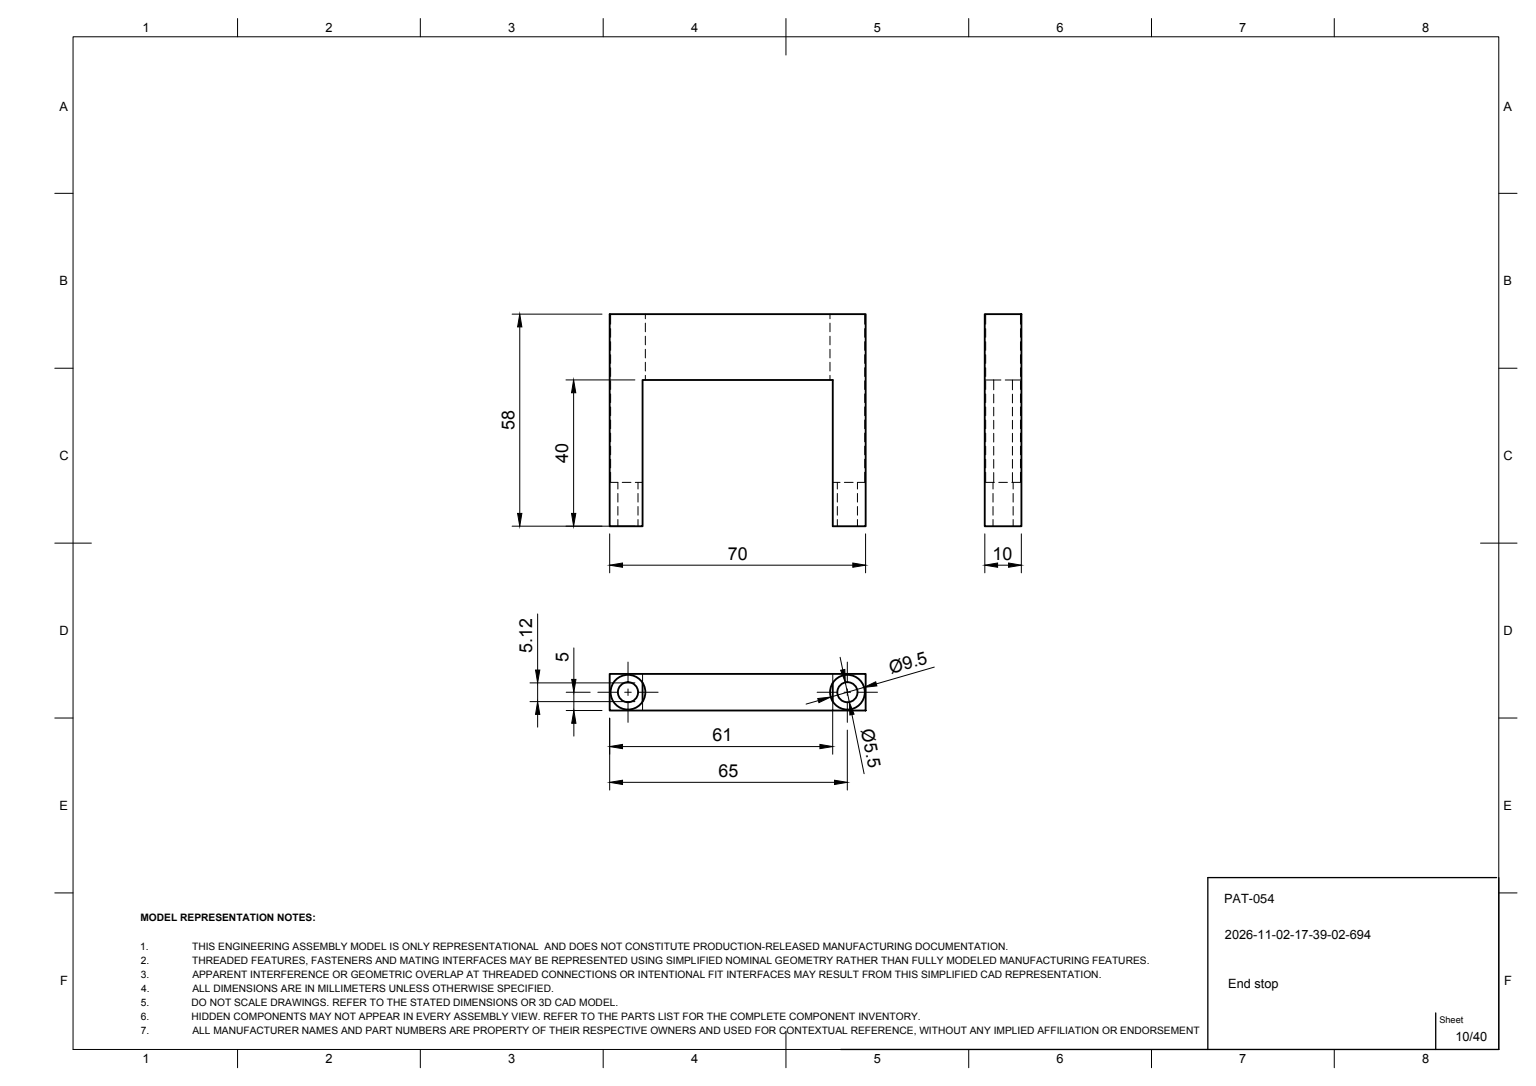
ISO-10303-21;
HEADER;
/* Generated by software containing ST-Developer
 * from STEP Tools, Inc. (www.steptools.com) 
 */

FILE_DESCRIPTION(
/* description */ ('PAT-054'),
/* implementation_level */ '2;1');

FILE_NAME(
/* name */ 'End stop.step',
/* time_stamp */ '2026-10-29T16:38:13-07:00',
/* author */ (''),
/* organization */ (''),
/* preprocessor_version */ 'ST-DEVELOPER v20.2',
/* originating_system */ 'Autodesk Translation Framework v15.17.0.0',
/* authorisation */ '');

FILE_SCHEMA (('AUTOMOTIVE_DESIGN { 1 0 10303 214 3 1 1 }'));
ENDSEC;

DATA;
#10=MECHANICAL_DESIGN_GEOMETRIC_PRESENTATION_REPRESENTATION('',(#905),#33981);
#817=SHAPE_REPRESENTATION_RELATIONSHIP('SRR','None',#34190,#861);
#861=ADVANCED_BREP_SHAPE_REPRESENTATION('',(#964),#33938);
#905=STYLED_ITEM('',(#34510),#964);
#964=MANIFOLD_SOLID_BREP('Body1',#13016);
#1104=FACE_BOUND('',#2486,.T.);
#1105=FACE_BOUND('',#2489,.T.);
#1106=FACE_BOUND('',#2498,.T.);
#1107=FACE_BOUND('',#2503,.T.);
#1108=FACE_BOUND('',#2504,.T.);
#1109=FACE_BOUND('',#2506,.T.);
#1269=PLANE('',#13771);
#1270=PLANE('',#13778);
#1271=PLANE('',#13785);
#1272=PLANE('',#13786);
#1273=PLANE('',#13791);
#1274=PLANE('',#13792);
#1275=PLANE('',#13793);
#1276=PLANE('',#13794);
#1277=PLANE('',#13795);
#1278=PLANE('',#13796);
#1279=PLANE('',#13797);
#1280=PLANE('',#13798);
#1670=FACE_OUTER_BOUND('',#2485,.T.);
#1671=FACE_OUTER_BOUND('',#2487,.T.);
#1672=FACE_OUTER_BOUND('',#2488,.T.);
#1673=FACE_OUTER_BOUND('',#2490,.T.);
#1674=FACE_OUTER_BOUND('',#2491,.T.);
#1675=FACE_OUTER_BOUND('',#2492,.T.);
#1676=FACE_OUTER_BOUND('',#2493,.T.);
#1677=FACE_OUTER_BOUND('',#2494,.T.);
#1678=FACE_OUTER_BOUND('',#2495,.T.);
#1679=FACE_OUTER_BOUND('',#2496,.T.);
#1680=FACE_OUTER_BOUND('',#2497,.T.);
#1681=FACE_OUTER_BOUND('',#2499,.T.);
#1682=FACE_OUTER_BOUND('',#2500,.T.);
#1683=FACE_OUTER_BOUND('',#2501,.T.);
#1684=FACE_OUTER_BOUND('',#2502,.T.);
#1685=FACE_OUTER_BOUND('',#2505,.T.);
#2485=EDGE_LOOP('',(#8915,#8916,#8917));
#2486=EDGE_LOOP('',(#8918));
#2487=EDGE_LOOP('',(#8919,#8920,#8921,#8922,#8923,#8924,#8925,#8926));
#2488=EDGE_LOOP('',(#8927,#8928,#8929));
#2489=EDGE_LOOP('',(#8930));
#2490=EDGE_LOOP('',(#8931,#8932,#8933,#8934,#8935,#8936,#8937,#8938));
#2491=EDGE_LOOP('',(#8939,#8940,#8941,#8942,#8943,#8944,#8945,#8946));
#2492=EDGE_LOOP('',(#8947,#8948,#8949,#8950,#8951,#8952,#8953,#8954));
#2493=EDGE_LOOP('',(#8955,#8956,#8957,#8958));
#2494=EDGE_LOOP('',(#8959,#8960,#8961,#8962));
#2495=EDGE_LOOP('',(#8963,#8964,#8965,#8966,#8967,#8968,#8969,#8970));
#2496=EDGE_LOOP('',(#8971,#8972,#8973,#8974,#8975,#8976,#8977,#8978));
#2497=EDGE_LOOP('',(#8979,#8980,#8981,#8982));
#2498=EDGE_LOOP('',(#8983));
#2499=EDGE_LOOP('',(#8984,#8985,#8986,#8987));
#2500=EDGE_LOOP('',(#8988,#8989,#8990,#8991));
#2501=EDGE_LOOP('',(#8992,#8993,#8994,#8995,#8996,#8997,#8998,#8999));
#2502=EDGE_LOOP('',(#9000,#9001,#9002,#9003));
#2503=EDGE_LOOP('',(#9004));
#2504=EDGE_LOOP('',(#9005));
#2505=EDGE_LOOP('',(#9006,#9007,#9008,#9009));
#2506=EDGE_LOOP('',(#9010));
#3342=LINE('',#18948,#4276);
#3343=LINE('',#18956,#4277);
#3344=LINE('',#18959,#4278);
#3345=LINE('',#18961,#4279);
#3346=LINE('',#18966,#4280);
#3347=LINE('',#18974,#4281);
#3348=LINE('',#18977,#4282);
#3349=LINE('',#18979,#4283);
#3350=LINE('',#18983,#4284);
#3351=LINE('',#18985,#4285);
#3352=LINE('',#18987,#4286);
#3353=LINE('',#18989,#4287);
#3354=LINE('',#18990,#4288);
#3355=LINE('',#18993,#4289);
#3356=LINE('',#18995,#4290);
#3357=LINE('',#18997,#4291);
#3358=LINE('',#18999,#4292);
#3359=LINE('',#19000,#4293);
#3360=LINE('',#19004,#4294);
#3361=LINE('',#19008,#4295);
#3362=LINE('',#19010,#4296);
#3363=LINE('',#19011,#4297);
#3364=LINE('',#19014,#4298);
#3365=LINE('',#19016,#4299);
#3366=LINE('',#19018,#4300);
#3367=LINE('',#19020,#4301);
#3368=LINE('',#19021,#4302);
#3369=LINE('',#19024,#4303);
#3370=LINE('',#19025,#4304);
#3371=LINE('',#19028,#4305);
#3372=LINE('',#19029,#4306);
#3373=LINE('',#19032,#4307);
#3374=LINE('',#19034,#4308);
#3375=LINE('',#19035,#4309);
#3376=LINE('',#19037,#4310);
#3377=LINE('',#19038,#4311);
#4276=VECTOR('',#15421,1.);
#4277=VECTOR('',#15430,1.);
#4278=VECTOR('',#15433,1.);
#4279=VECTOR('',#15434,0.475);
#4280=VECTOR('',#15439,1.);
#4281=VECTOR('',#15448,1.);
#4282=VECTOR('',#15451,1.);
#4283=VECTOR('',#15452,0.475);
#4284=VECTOR('',#15457,1.);
#4285=VECTOR('',#15458,1.);
#4286=VECTOR('',#15459,1.);
#4287=VECTOR('',#15460,1.);
#4288=VECTOR('',#15461,1.);
#4289=VECTOR('',#15464,1.);
#4290=VECTOR('',#15465,1.);
#4291=VECTOR('',#15466,1.);
#4292=VECTOR('',#15467,1.);
#4293=VECTOR('',#15468,1.);
#4294=VECTOR('',#15473,0.275);
#4295=VECTOR('',#15478,0.275);
#4296=VECTOR('',#15481,1.);
#4297=VECTOR('',#15482,1.);
#4298=VECTOR('',#15485,1.);
#4299=VECTOR('',#15486,1.);
#4300=VECTOR('',#15487,1.);
#4301=VECTOR('',#15488,1.);
#4302=VECTOR('',#15489,1.);
#4303=VECTOR('',#15492,1.);
#4304=VECTOR('',#15493,1.);
#4305=VECTOR('',#15496,1.);
#4306=VECTOR('',#15497,1.);
#4307=VECTOR('',#15500,1.);
#4308=VECTOR('',#15501,1.);
#4309=VECTOR('',#15502,1.);
#4310=VECTOR('',#15505,1.);
#4311=VECTOR('',#15506,1.);
#5213=CIRCLE('',#13772,0.475);
#5214=CIRCLE('',#13773,0.475);
#5215=CIRCLE('',#13774,0.275);
#5216=CIRCLE('',#13776,0.475);
#5217=CIRCLE('',#13777,0.475);
#5218=CIRCLE('',#13779,0.475);
#5219=CIRCLE('',#13780,0.475);
#5220=CIRCLE('',#13781,0.275);
#5221=CIRCLE('',#13783,0.475);
#5222=CIRCLE('',#13784,0.475);
#5223=CIRCLE('',#13788,0.275);
#5224=CIRCLE('',#13790,0.275);
#5712=VERTEX_POINT('',#18946);
#5713=VERTEX_POINT('',#18947);
#5714=VERTEX_POINT('',#18949);
#5715=VERTEX_POINT('',#18952);
#5716=VERTEX_POINT('',#18955);
#5717=VERTEX_POINT('',#18957);
#5718=VERTEX_POINT('',#18960);
#5719=VERTEX_POINT('',#18964);
#5720=VERTEX_POINT('',#18965);
#5721=VERTEX_POINT('',#18967);
#5722=VERTEX_POINT('',#18970);
#5723=VERTEX_POINT('',#18973);
#5724=VERTEX_POINT('',#18975);
#5725=VERTEX_POINT('',#18978);
#5726=VERTEX_POINT('',#18982);
#5727=VERTEX_POINT('',#18984);
#5728=VERTEX_POINT('',#18986);
#5729=VERTEX_POINT('',#18988);
#5730=VERTEX_POINT('',#18992);
#5731=VERTEX_POINT('',#18994);
#5732=VERTEX_POINT('',#18996);
#5733=VERTEX_POINT('',#18998);
#5734=VERTEX_POINT('',#19002);
#5735=VERTEX_POINT('',#19006);
#5736=VERTEX_POINT('',#19013);
#5737=VERTEX_POINT('',#19015);
#5738=VERTEX_POINT('',#19017);
#5739=VERTEX_POINT('',#19019);
#5740=VERTEX_POINT('',#19023);
#5741=VERTEX_POINT('',#19027);
#5742=VERTEX_POINT('',#19031);
#5743=VERTEX_POINT('',#19033);
#6957=EDGE_CURVE('',#5712,#5713,#3342,.T.);
#6958=EDGE_CURVE('',#5712,#5714,#5213,.T.);
#6959=EDGE_CURVE('',#5714,#5713,#5214,.T.);
#6960=EDGE_CURVE('',#5715,#5715,#5215,.T.);
#6961=EDGE_CURVE('',#5716,#5712,#3343,.T.);
#6962=EDGE_CURVE('',#5717,#5716,#5216,.T.);
#6963=EDGE_CURVE('',#5713,#5717,#3344,.T.);
#6964=EDGE_CURVE('',#5714,#5718,#3345,.T.);
#6965=EDGE_CURVE('',#5718,#5718,#5217,.T.);
#6966=EDGE_CURVE('',#5719,#5720,#3346,.T.);
#6967=EDGE_CURVE('',#5719,#5721,#5218,.T.);
#6968=EDGE_CURVE('',#5721,#5720,#5219,.T.);
#6969=EDGE_CURVE('',#5722,#5722,#5220,.T.);
#6970=EDGE_CURVE('',#5723,#5719,#3347,.T.);
#6971=EDGE_CURVE('',#5724,#5723,#5221,.T.);
#6972=EDGE_CURVE('',#5720,#5724,#3348,.T.);
#6973=EDGE_CURVE('',#5721,#5725,#3349,.T.);
#6974=EDGE_CURVE('',#5725,#5725,#5222,.T.);
#6975=EDGE_CURVE('',#5717,#5726,#3350,.T.);
#6976=EDGE_CURVE('',#5727,#5726,#3351,.T.);
#6977=EDGE_CURVE('',#5728,#5727,#3352,.T.);
#6978=EDGE_CURVE('',#5729,#5728,#3353,.T.);
#6979=EDGE_CURVE('',#5729,#5716,#3354,.T.);
#6980=EDGE_CURVE('',#5730,#5724,#3355,.T.);
#6981=EDGE_CURVE('',#5731,#5730,#3356,.T.);
#6982=EDGE_CURVE('',#5732,#5731,#3357,.T.);
#6983=EDGE_CURVE('',#5733,#5732,#3358,.T.);
#6984=EDGE_CURVE('',#5723,#5733,#3359,.T.);
#6985=EDGE_CURVE('',#5734,#5734,#5223,.T.);
#6986=EDGE_CURVE('',#5734,#5715,#3360,.T.);
#6987=EDGE_CURVE('',#5735,#5735,#5224,.T.);
#6988=EDGE_CURVE('',#5735,#5722,#3361,.T.);
#6989=EDGE_CURVE('',#5730,#5729,#3362,.T.);
#6990=EDGE_CURVE('',#5726,#5733,#3363,.T.);
#6991=EDGE_CURVE('',#5732,#5736,#3364,.T.);
#6992=EDGE_CURVE('',#5736,#5737,#3365,.T.);
#6993=EDGE_CURVE('',#5738,#5737,#3366,.T.);
#6994=EDGE_CURVE('',#5739,#5738,#3367,.T.);
#6995=EDGE_CURVE('',#5739,#5727,#3368,.T.);
#6996=EDGE_CURVE('',#5740,#5731,#3369,.T.);
#6997=EDGE_CURVE('',#5736,#5740,#3370,.T.);
#6998=EDGE_CURVE('',#5740,#5741,#3371,.T.);
#6999=EDGE_CURVE('',#5737,#5741,#3372,.T.);
#7000=EDGE_CURVE('',#5742,#5739,#3373,.T.);
#7001=EDGE_CURVE('',#5743,#5738,#3374,.T.);
#7002=EDGE_CURVE('',#5742,#5743,#3375,.T.);
#7003=EDGE_CURVE('',#5728,#5742,#3376,.T.);
#7004=EDGE_CURVE('',#5741,#5743,#3377,.T.);
#8915=ORIENTED_EDGE('',*,*,#6957,.F.);
#8916=ORIENTED_EDGE('',*,*,#6958,.T.);
#8917=ORIENTED_EDGE('',*,*,#6959,.T.);
#8918=ORIENTED_EDGE('',*,*,#6960,.F.);
#8919=ORIENTED_EDGE('',*,*,#6961,.F.);
#8920=ORIENTED_EDGE('',*,*,#6962,.F.);
#8921=ORIENTED_EDGE('',*,*,#6963,.F.);
#8922=ORIENTED_EDGE('',*,*,#6959,.F.);
#8923=ORIENTED_EDGE('',*,*,#6964,.T.);
#8924=ORIENTED_EDGE('',*,*,#6965,.F.);
#8925=ORIENTED_EDGE('',*,*,#6964,.F.);
#8926=ORIENTED_EDGE('',*,*,#6958,.F.);
#8927=ORIENTED_EDGE('',*,*,#6966,.F.);
#8928=ORIENTED_EDGE('',*,*,#6967,.T.);
#8929=ORIENTED_EDGE('',*,*,#6968,.T.);
#8930=ORIENTED_EDGE('',*,*,#6969,.F.);
#8931=ORIENTED_EDGE('',*,*,#6970,.F.);
#8932=ORIENTED_EDGE('',*,*,#6971,.F.);
#8933=ORIENTED_EDGE('',*,*,#6972,.F.);
#8934=ORIENTED_EDGE('',*,*,#6968,.F.);
#8935=ORIENTED_EDGE('',*,*,#6973,.T.);
#8936=ORIENTED_EDGE('',*,*,#6974,.F.);
#8937=ORIENTED_EDGE('',*,*,#6973,.F.);
#8938=ORIENTED_EDGE('',*,*,#6967,.F.);
#8939=ORIENTED_EDGE('',*,*,#6961,.T.);
#8940=ORIENTED_EDGE('',*,*,#6957,.T.);
#8941=ORIENTED_EDGE('',*,*,#6963,.T.);
#8942=ORIENTED_EDGE('',*,*,#6975,.T.);
#8943=ORIENTED_EDGE('',*,*,#6976,.F.);
#8944=ORIENTED_EDGE('',*,*,#6977,.F.);
#8945=ORIENTED_EDGE('',*,*,#6978,.F.);
#8946=ORIENTED_EDGE('',*,*,#6979,.T.);
#8947=ORIENTED_EDGE('',*,*,#6970,.T.);
#8948=ORIENTED_EDGE('',*,*,#6966,.T.);
#8949=ORIENTED_EDGE('',*,*,#6972,.T.);
#8950=ORIENTED_EDGE('',*,*,#6980,.F.);
#8951=ORIENTED_EDGE('',*,*,#6981,.F.);
#8952=ORIENTED_EDGE('',*,*,#6982,.F.);
#8953=ORIENTED_EDGE('',*,*,#6983,.F.);
#8954=ORIENTED_EDGE('',*,*,#6984,.F.);
#8955=ORIENTED_EDGE('',*,*,#6985,.F.);
#8956=ORIENTED_EDGE('',*,*,#6986,.T.);
#8957=ORIENTED_EDGE('',*,*,#6960,.T.);
#8958=ORIENTED_EDGE('',*,*,#6986,.F.);
#8959=ORIENTED_EDGE('',*,*,#6987,.F.);
#8960=ORIENTED_EDGE('',*,*,#6988,.T.);
#8961=ORIENTED_EDGE('',*,*,#6969,.T.);
#8962=ORIENTED_EDGE('',*,*,#6988,.F.);
#8963=ORIENTED_EDGE('',*,*,#6962,.T.);
#8964=ORIENTED_EDGE('',*,*,#6979,.F.);
#8965=ORIENTED_EDGE('',*,*,#6989,.F.);
#8966=ORIENTED_EDGE('',*,*,#6980,.T.);
#8967=ORIENTED_EDGE('',*,*,#6971,.T.);
#8968=ORIENTED_EDGE('',*,*,#6984,.T.);
#8969=ORIENTED_EDGE('',*,*,#6990,.F.);
#8970=ORIENTED_EDGE('',*,*,#6975,.F.);
#8971=ORIENTED_EDGE('',*,*,#6976,.T.);
#8972=ORIENTED_EDGE('',*,*,#6990,.T.);
#8973=ORIENTED_EDGE('',*,*,#6983,.T.);
#8974=ORIENTED_EDGE('',*,*,#6991,.T.);
#8975=ORIENTED_EDGE('',*,*,#6992,.T.);
#8976=ORIENTED_EDGE('',*,*,#6993,.F.);
#8977=ORIENTED_EDGE('',*,*,#6994,.F.);
#8978=ORIENTED_EDGE('',*,*,#6995,.T.);
#8979=ORIENTED_EDGE('',*,*,#6982,.T.);
#8980=ORIENTED_EDGE('',*,*,#6996,.F.);
#8981=ORIENTED_EDGE('',*,*,#6997,.F.);
#8982=ORIENTED_EDGE('',*,*,#6991,.F.);
#8983=ORIENTED_EDGE('',*,*,#6987,.T.);
#8984=ORIENTED_EDGE('',*,*,#6997,.T.);
#8985=ORIENTED_EDGE('',*,*,#6998,.T.);
#8986=ORIENTED_EDGE('',*,*,#6999,.F.);
#8987=ORIENTED_EDGE('',*,*,#6992,.F.);
#8988=ORIENTED_EDGE('',*,*,#7000,.T.);
#8989=ORIENTED_EDGE('',*,*,#6994,.T.);
#8990=ORIENTED_EDGE('',*,*,#7001,.F.);
#8991=ORIENTED_EDGE('',*,*,#7002,.F.);
#8992=ORIENTED_EDGE('',*,*,#6978,.T.);
#8993=ORIENTED_EDGE('',*,*,#7003,.T.);
#8994=ORIENTED_EDGE('',*,*,#7002,.T.);
#8995=ORIENTED_EDGE('',*,*,#7004,.F.);
#8996=ORIENTED_EDGE('',*,*,#6998,.F.);
#8997=ORIENTED_EDGE('',*,*,#6996,.T.);
#8998=ORIENTED_EDGE('',*,*,#6981,.T.);
#8999=ORIENTED_EDGE('',*,*,#6989,.T.);
#9000=ORIENTED_EDGE('',*,*,#7004,.T.);
#9001=ORIENTED_EDGE('',*,*,#7001,.T.);
#9002=ORIENTED_EDGE('',*,*,#6993,.T.);
#9003=ORIENTED_EDGE('',*,*,#6999,.T.);
#9004=ORIENTED_EDGE('',*,*,#6965,.T.);
#9005=ORIENTED_EDGE('',*,*,#6974,.T.);
#9006=ORIENTED_EDGE('',*,*,#6977,.T.);
#9007=ORIENTED_EDGE('',*,*,#6995,.F.);
#9008=ORIENTED_EDGE('',*,*,#7000,.F.);
#9009=ORIENTED_EDGE('',*,*,#7003,.F.);
#9010=ORIENTED_EDGE('',*,*,#6985,.T.);
#12033=CYLINDRICAL_SURFACE('',#13775,0.475);
#12034=CYLINDRICAL_SURFACE('',#13782,0.475);
#12035=CYLINDRICAL_SURFACE('',#13787,0.275);
#12036=CYLINDRICAL_SURFACE('',#13789,0.275);
#12382=ADVANCED_FACE('',(#1670,#1104),#1269,.T.);
#12383=ADVANCED_FACE('',(#1671),#12033,.F.);
#12384=ADVANCED_FACE('',(#1672,#1105),#1270,.T.);
#12385=ADVANCED_FACE('',(#1673),#12034,.F.);
#12386=ADVANCED_FACE('',(#1674),#1271,.F.);
#12387=ADVANCED_FACE('',(#1675),#1272,.F.);
#12388=ADVANCED_FACE('',(#1676),#12035,.F.);
#12389=ADVANCED_FACE('',(#1677),#12036,.F.);
#12390=ADVANCED_FACE('',(#1678),#1273,.F.);
#12391=ADVANCED_FACE('',(#1679),#1274,.T.);
#12392=ADVANCED_FACE('',(#1680,#1106),#1275,.F.);
#12393=ADVANCED_FACE('',(#1681),#1276,.T.);
#12394=ADVANCED_FACE('',(#1682),#1277,.T.);
#12395=ADVANCED_FACE('',(#1683),#1278,.T.);
#12396=ADVANCED_FACE('',(#1684,#1107,#1108),#1279,.T.);
#12397=ADVANCED_FACE('',(#1685,#1109),#1280,.F.);
#13016=CLOSED_SHELL('',(#12382,#12383,#12384,#12385,#12386,#12387,#12388,
#12389,#12390,#12391,#12392,#12393,#12394,#12395,#12396,#12397));
#13770=AXIS2_PLACEMENT_3D('',#18944,#15417,#15418);
#13771=AXIS2_PLACEMENT_3D('',#18945,#15419,#15420);
#13772=AXIS2_PLACEMENT_3D('',#18950,#15422,#15423);
#13773=AXIS2_PLACEMENT_3D('',#18951,#15424,#15425);
#13774=AXIS2_PLACEMENT_3D('',#18953,#15426,#15427);
#13775=AXIS2_PLACEMENT_3D('',#18954,#15428,#15429);
#13776=AXIS2_PLACEMENT_3D('',#18958,#15431,#15432);
#13777=AXIS2_PLACEMENT_3D('',#18962,#15435,#15436);
#13778=AXIS2_PLACEMENT_3D('',#18963,#15437,#15438);
#13779=AXIS2_PLACEMENT_3D('',#18968,#15440,#15441);
#13780=AXIS2_PLACEMENT_3D('',#18969,#15442,#15443);
#13781=AXIS2_PLACEMENT_3D('',#18971,#15444,#15445);
#13782=AXIS2_PLACEMENT_3D('',#18972,#15446,#15447);
#13783=AXIS2_PLACEMENT_3D('',#18976,#15449,#15450);
#13784=AXIS2_PLACEMENT_3D('',#18980,#15453,#15454);
#13785=AXIS2_PLACEMENT_3D('',#18981,#15455,#15456);
#13786=AXIS2_PLACEMENT_3D('',#18991,#15462,#15463);
#13787=AXIS2_PLACEMENT_3D('',#19001,#15469,#15470);
#13788=AXIS2_PLACEMENT_3D('',#19003,#15471,#15472);
#13789=AXIS2_PLACEMENT_3D('',#19005,#15474,#15475);
#13790=AXIS2_PLACEMENT_3D('',#19007,#15476,#15477);
#13791=AXIS2_PLACEMENT_3D('',#19009,#15479,#15480);
#13792=AXIS2_PLACEMENT_3D('',#19012,#15483,#15484);
#13793=AXIS2_PLACEMENT_3D('',#19022,#15490,#15491);
#13794=AXIS2_PLACEMENT_3D('',#19026,#15494,#15495);
#13795=AXIS2_PLACEMENT_3D('',#19030,#15498,#15499);
#13796=AXIS2_PLACEMENT_3D('',#19036,#15503,#15504);
#13797=AXIS2_PLACEMENT_3D('',#19039,#15507,#15508);
#13798=AXIS2_PLACEMENT_3D('',#19040,#15509,#15510);
#15417=DIRECTION('axis',(0.,0.,1.));
#15418=DIRECTION('refdir',(1.,0.,0.));
#15419=DIRECTION('center_axis',(0.,0.,1.));
#15420=DIRECTION('ref_axis',(1.,0.,0.));
#15421=DIRECTION('',(1.,0.,0.));
#15422=DIRECTION('center_axis',(0.,0.,1.));
#15423=DIRECTION('ref_axis',(1.,0.,0.));
#15424=DIRECTION('center_axis',(0.,0.,1.));
#15425=DIRECTION('ref_axis',(1.,0.,0.));
#15426=DIRECTION('center_axis',(0.,0.,1.));
#15427=DIRECTION('ref_axis',(1.,0.,0.));
#15428=DIRECTION('center_axis',(0.,0.,1.));
#15429=DIRECTION('ref_axis',(1.,0.,0.));
#15430=DIRECTION('',(0.,0.,-1.));
#15431=DIRECTION('center_axis',(0.,0.,1.));
#15432=DIRECTION('ref_axis',(1.,0.,0.));
#15433=DIRECTION('',(0.,0.,1.));
#15434=DIRECTION('',(0.,0.,1.));
#15435=DIRECTION('center_axis',(0.,0.,-1.));
#15436=DIRECTION('ref_axis',(1.,0.,0.));
#15437=DIRECTION('center_axis',(0.,0.,1.));
#15438=DIRECTION('ref_axis',(1.,0.,0.));
#15439=DIRECTION('',(-1.,0.,0.));
#15440=DIRECTION('center_axis',(0.,0.,1.));
#15441=DIRECTION('ref_axis',(1.,0.,0.));
#15442=DIRECTION('center_axis',(0.,0.,1.));
#15443=DIRECTION('ref_axis',(1.,0.,0.));
#15444=DIRECTION('center_axis',(0.,0.,1.));
#15445=DIRECTION('ref_axis',(1.,0.,0.));
#15446=DIRECTION('center_axis',(0.,0.,1.));
#15447=DIRECTION('ref_axis',(1.,0.,0.));
#15448=DIRECTION('',(0.,0.,-1.));
#15449=DIRECTION('center_axis',(0.,0.,1.));
#15450=DIRECTION('ref_axis',(1.,0.,0.));
#15451=DIRECTION('',(0.,0.,1.));
#15452=DIRECTION('',(0.,0.,1.));
#15453=DIRECTION('center_axis',(0.,0.,-1.));
#15454=DIRECTION('ref_axis',(1.,0.,0.));
#15455=DIRECTION('center_axis',(0.,-1.,0.));
#15456=DIRECTION('ref_axis',(0.,0.,-1.));
#15457=DIRECTION('',(1.,0.,0.));
#15458=DIRECTION('',(0.,0.,1.));
#15459=DIRECTION('',(1.,0.,0.));
#15460=DIRECTION('',(0.,0.,-1.));
#15461=DIRECTION('',(1.,0.,0.));
#15462=DIRECTION('center_axis',(0.,1.,0.));
#15463=DIRECTION('ref_axis',(0.,0.,1.));
#15464=DIRECTION('',(1.,0.,0.));
#15465=DIRECTION('',(0.,0.,1.));
#15466=DIRECTION('',(-1.,0.,0.));
#15467=DIRECTION('',(0.,0.,-1.));
#15468=DIRECTION('',(1.,0.,0.));
#15469=DIRECTION('center_axis',(0.,0.,1.));
#15470=DIRECTION('ref_axis',(1.,0.,0.));
#15471=DIRECTION('center_axis',(0.,0.,1.));
#15472=DIRECTION('ref_axis',(1.,0.,0.));
#15473=DIRECTION('',(0.,0.,1.));
#15474=DIRECTION('center_axis',(0.,0.,1.));
#15475=DIRECTION('ref_axis',(1.,0.,0.));
#15476=DIRECTION('center_axis',(0.,0.,1.));
#15477=DIRECTION('ref_axis',(1.,0.,0.));
#15478=DIRECTION('',(0.,0.,1.));
#15479=DIRECTION('center_axis',(0.,0.,1.));
#15480=DIRECTION('ref_axis',(0.,-1.,0.));
#15481=DIRECTION('',(0.,-1.,0.));
#15482=DIRECTION('',(0.,1.,0.));
#15483=DIRECTION('center_axis',(1.,0.,0.));
#15484=DIRECTION('ref_axis',(0.,1.,0.));
#15485=DIRECTION('',(0.,1.,0.));
#15486=DIRECTION('',(0.,0.,1.));
#15487=DIRECTION('',(0.,1.,0.));
#15488=DIRECTION('',(0.,0.,1.));
#15489=DIRECTION('',(0.,1.,0.));
#15490=DIRECTION('center_axis',(0.,0.,1.));
#15491=DIRECTION('ref_axis',(1.,0.,0.));
#15492=DIRECTION('',(0.,-1.,0.));
#15493=DIRECTION('',(-1.,0.,0.));
#15494=DIRECTION('center_axis',(0.,1.,0.));
#15495=DIRECTION('ref_axis',(-1.,0.,0.));
#15496=DIRECTION('',(0.,0.,1.));
#15497=DIRECTION('',(-1.,0.,0.));
#15498=DIRECTION('center_axis',(0.,-1.,0.));
#15499=DIRECTION('ref_axis',(1.,0.,0.));
#15500=DIRECTION('',(1.,0.,0.));
#15501=DIRECTION('',(1.,0.,0.));
#15502=DIRECTION('',(0.,0.,1.));
#15503=DIRECTION('center_axis',(-1.,0.,0.));
#15504=DIRECTION('ref_axis',(0.,-1.,0.));
#15505=DIRECTION('',(0.,-1.,0.));
#15506=DIRECTION('',(0.,-1.,0.));
#15507=DIRECTION('center_axis',(0.,0.,1.));
#15508=DIRECTION('ref_axis',(1.,0.,0.));
#15509=DIRECTION('center_axis',(0.,0.,1.));
#15510=DIRECTION('ref_axis',(1.,0.,0.));
#18944=CARTESIAN_POINT('',(0.,0.,0.));
#18945=CARTESIAN_POINT('Origin',(4.7,-9.,2.4));
#18946=CARTESIAN_POINT('',(4.44382623085101,-8.6,2.4));
#18947=CARTESIAN_POINT('',(4.95617376914899,-8.6,2.4));
#18948=CARTESIAN_POINT('',(4.4,-8.6,2.4));
#18949=CARTESIAN_POINT('',(4.225,-9.,2.4));
#18950=CARTESIAN_POINT('Origin',(4.7,-9.,2.4));
#18951=CARTESIAN_POINT('Origin',(4.7,-9.,2.4));
#18952=CARTESIAN_POINT('',(4.425,-9.,2.4));
#18953=CARTESIAN_POINT('Origin',(4.7,-9.,2.4));
#18954=CARTESIAN_POINT('Origin',(4.7,-9.,2.4));
#18955=CARTESIAN_POINT('',(4.44382623085101,-8.6,5.2));
#18956=CARTESIAN_POINT('',(4.44382623085101,-8.6,2.4));
#18957=CARTESIAN_POINT('',(4.95617376914899,-8.6,5.2));
#18958=CARTESIAN_POINT('Origin',(4.7,-9.,5.2));
#18959=CARTESIAN_POINT('',(4.95617376914899,-8.6,2.4));
#18960=CARTESIAN_POINT('',(4.225,-9.,7.));
#18961=CARTESIAN_POINT('',(4.225,-9.,2.4));
#18962=CARTESIAN_POINT('Origin',(4.7,-9.,7.));
#18963=CARTESIAN_POINT('Origin',(4.7,-3.,2.4));
#18964=CARTESIAN_POINT('',(4.95617376914899,-3.4,2.4));
#18965=CARTESIAN_POINT('',(4.44382623085101,-3.4,2.4));
#18966=CARTESIAN_POINT('',(4.4,-3.4,2.4));
#18967=CARTESIAN_POINT('',(4.225,-3.,2.4));
#18968=CARTESIAN_POINT('Origin',(4.7,-3.,2.4));
#18969=CARTESIAN_POINT('Origin',(4.7,-3.,2.4));
#18970=CARTESIAN_POINT('',(4.425,-3.,2.4));
#18971=CARTESIAN_POINT('Origin',(4.7,-3.,2.4));
#18972=CARTESIAN_POINT('Origin',(4.7,-3.,2.4));
#18973=CARTESIAN_POINT('',(4.95617376914899,-3.4,5.2));
#18974=CARTESIAN_POINT('',(4.95617376914899,-3.4,2.4));
#18975=CARTESIAN_POINT('',(4.44382623085101,-3.4,5.2));
#18976=CARTESIAN_POINT('Origin',(4.7,-3.,5.2));
#18977=CARTESIAN_POINT('',(4.44382623085101,-3.4,2.4));
#18978=CARTESIAN_POINT('',(4.225,-3.,7.));
#18979=CARTESIAN_POINT('',(4.225,-3.,2.4));
#18980=CARTESIAN_POINT('Origin',(4.7,-3.,7.));
#18981=CARTESIAN_POINT('Origin',(4.1,-8.6,5.2));
#18982=CARTESIAN_POINT('',(5.2,-8.6,5.2));
#18983=CARTESIAN_POINT('',(4.1,-8.6,5.2));
#18984=CARTESIAN_POINT('',(5.2,-8.6,1.2));
#18985=CARTESIAN_POINT('',(5.2,-8.6,3.2));
#18986=CARTESIAN_POINT('',(4.2,-8.6,1.2));
#18987=CARTESIAN_POINT('',(4.4,-8.6,1.2));
#18988=CARTESIAN_POINT('',(4.2,-8.6,5.2));
#18989=CARTESIAN_POINT('',(4.2,-8.6,3.2));
#18990=CARTESIAN_POINT('',(4.1,-8.6,5.2));
#18991=CARTESIAN_POINT('Origin',(4.1,-3.4,1.2));
#18992=CARTESIAN_POINT('',(4.2,-3.4,5.2));
#18993=CARTESIAN_POINT('',(4.1,-3.4,5.2));
#18994=CARTESIAN_POINT('',(4.2,-3.4,1.2));
#18995=CARTESIAN_POINT('',(4.2,-3.4,1.2));
#18996=CARTESIAN_POINT('',(5.2,-3.4,1.2));
#18997=CARTESIAN_POINT('',(4.4,-3.4,1.2));
#18998=CARTESIAN_POINT('',(5.2,-3.4,5.2));
#18999=CARTESIAN_POINT('',(5.2,-3.4,1.2));
#19000=CARTESIAN_POINT('',(4.1,-3.4,5.2));
#19001=CARTESIAN_POINT('Origin',(4.7,-9.,1.1));
#19002=CARTESIAN_POINT('',(4.425,-9.,1.2));
#19003=CARTESIAN_POINT('Origin',(4.7,-9.,1.2));
#19004=CARTESIAN_POINT('',(4.425,-9.,1.1));
#19005=CARTESIAN_POINT('Origin',(4.7,-3.,1.1));
#19006=CARTESIAN_POINT('',(4.425,-3.,1.2));
#19007=CARTESIAN_POINT('Origin',(4.7,-3.,1.2));
#19008=CARTESIAN_POINT('',(4.425,-3.,1.1));
#19009=CARTESIAN_POINT('Origin',(4.1,-3.4,5.2));
#19010=CARTESIAN_POINT('',(4.2,-2.95,5.2));
#19011=CARTESIAN_POINT('',(5.2,-6.45,5.2));
#19012=CARTESIAN_POINT('Origin',(5.2,-9.5,1.2));
#19013=CARTESIAN_POINT('',(5.2,-2.5,1.2));
#19014=CARTESIAN_POINT('',(5.2,-9.5,1.2));
#19015=CARTESIAN_POINT('',(5.2,-2.5,7.));
#19016=CARTESIAN_POINT('',(5.2,-2.5,1.2));
#19017=CARTESIAN_POINT('',(5.2,-9.5,7.));
#19018=CARTESIAN_POINT('',(5.2,-9.5,7.));
#19019=CARTESIAN_POINT('',(5.2,-9.5,1.2));
#19020=CARTESIAN_POINT('',(5.2,-9.5,1.2));
#19021=CARTESIAN_POINT('',(5.2,-9.5,1.2));
#19022=CARTESIAN_POINT('Origin',(4.7,-6.,1.2));
#19023=CARTESIAN_POINT('',(4.2,-2.5,1.2));
#19024=CARTESIAN_POINT('',(4.2,-2.5,1.2));
#19025=CARTESIAN_POINT('',(5.2,-2.5,1.2));
#19026=CARTESIAN_POINT('Origin',(5.2,-2.5,1.2));
#19027=CARTESIAN_POINT('',(4.2,-2.5,7.));
#19028=CARTESIAN_POINT('',(4.2,-2.5,1.2));
#19029=CARTESIAN_POINT('',(5.2,-2.5,7.));
#19030=CARTESIAN_POINT('Origin',(4.2,-9.5,1.2));
#19031=CARTESIAN_POINT('',(4.2,-9.5,1.2));
#19032=CARTESIAN_POINT('',(4.2,-9.5,1.2));
#19033=CARTESIAN_POINT('',(4.2,-9.5,7.));
#19034=CARTESIAN_POINT('',(4.2,-9.5,7.));
#19035=CARTESIAN_POINT('',(4.2,-9.5,1.2));
#19036=CARTESIAN_POINT('Origin',(4.2,-2.5,1.2));
#19037=CARTESIAN_POINT('',(4.2,-2.5,1.2));
#19038=CARTESIAN_POINT('',(4.2,-2.5,7.));
#19039=CARTESIAN_POINT('Origin',(4.7,-6.,7.));
#19040=CARTESIAN_POINT('Origin',(4.7,-6.,1.2));
#33886=UNCERTAINTY_MEASURE_WITH_UNIT(LENGTH_MEASURE(0.001),#33982,
'DISTANCE_ACCURACY_VALUE',
'Maximum model space distance between geometric entities at asserted c
onnectivities');
#33929=UNCERTAINTY_MEASURE_WITH_UNIT(LENGTH_MEASURE(0.001),#33982,
'DISTANCE_ACCURACY_VALUE',
'Maximum model space distance between geometric entities at asserted c
onnectivities');
#33938=(
GEOMETRIC_REPRESENTATION_CONTEXT(3)
GLOBAL_UNCERTAINTY_ASSIGNED_CONTEXT((#33886))
GLOBAL_UNIT_ASSIGNED_CONTEXT((#33982,#33984,#33985))
REPRESENTATION_CONTEXT('','3D')
);
#33981=(
GEOMETRIC_REPRESENTATION_CONTEXT(3)
GLOBAL_UNCERTAINTY_ASSIGNED_CONTEXT((#33929))
GLOBAL_UNIT_ASSIGNED_CONTEXT((#33982,#33984,#33985))
REPRESENTATION_CONTEXT('','3D')
);
#33982=(
LENGTH_UNIT()
NAMED_UNIT(*)
SI_UNIT(.CENTI.,.METRE.)
);
#33984=(
NAMED_UNIT(*)
PLANE_ANGLE_UNIT()
SI_UNIT($,.RADIAN.)
);
#33985=(
NAMED_UNIT(*)
SI_UNIT($,.STERADIAN.)
SOLID_ANGLE_UNIT()
);
#33994=SHAPE_DEFINITION_REPRESENTATION(#34045,#34190);
#34045=PRODUCT_DEFINITION_SHAPE('',$,#34242);
#34190=SHAPE_REPRESENTATION('',(#13770),#33938);
#34233=PRODUCT_DEFINITION_CONTEXT('part definition',#34388,'design');
#34242=PRODUCT_DEFINITION('End stop','End stop',#34293,#34233);
#34293=PRODUCT_DEFINITION_FORMATION('',$,#34398);
#34388=APPLICATION_CONTEXT(
'Core Data for Automotive Mechanical Design Process');
#34389=PRODUCT_CONTEXT('part definition',#34388,'mechanical');
#34398=PRODUCT('End stop','End stop','End stop',(#34389));
#34504=COLOUR_RGB('Sky Blue',0.24,0.69,0.87);
#34505=FILL_AREA_STYLE_COLOUR('',#34504);
#34506=FILL_AREA_STYLE('',(#34505));
#34507=SURFACE_STYLE_FILL_AREA(#34506);
#34508=SURFACE_SIDE_STYLE('',(#34507));
#34509=SURFACE_STYLE_USAGE(.BOTH.,#34508);
#34510=PRESENTATION_STYLE_ASSIGNMENT((#34509));
ENDSEC;
END-ISO-10303-21;
